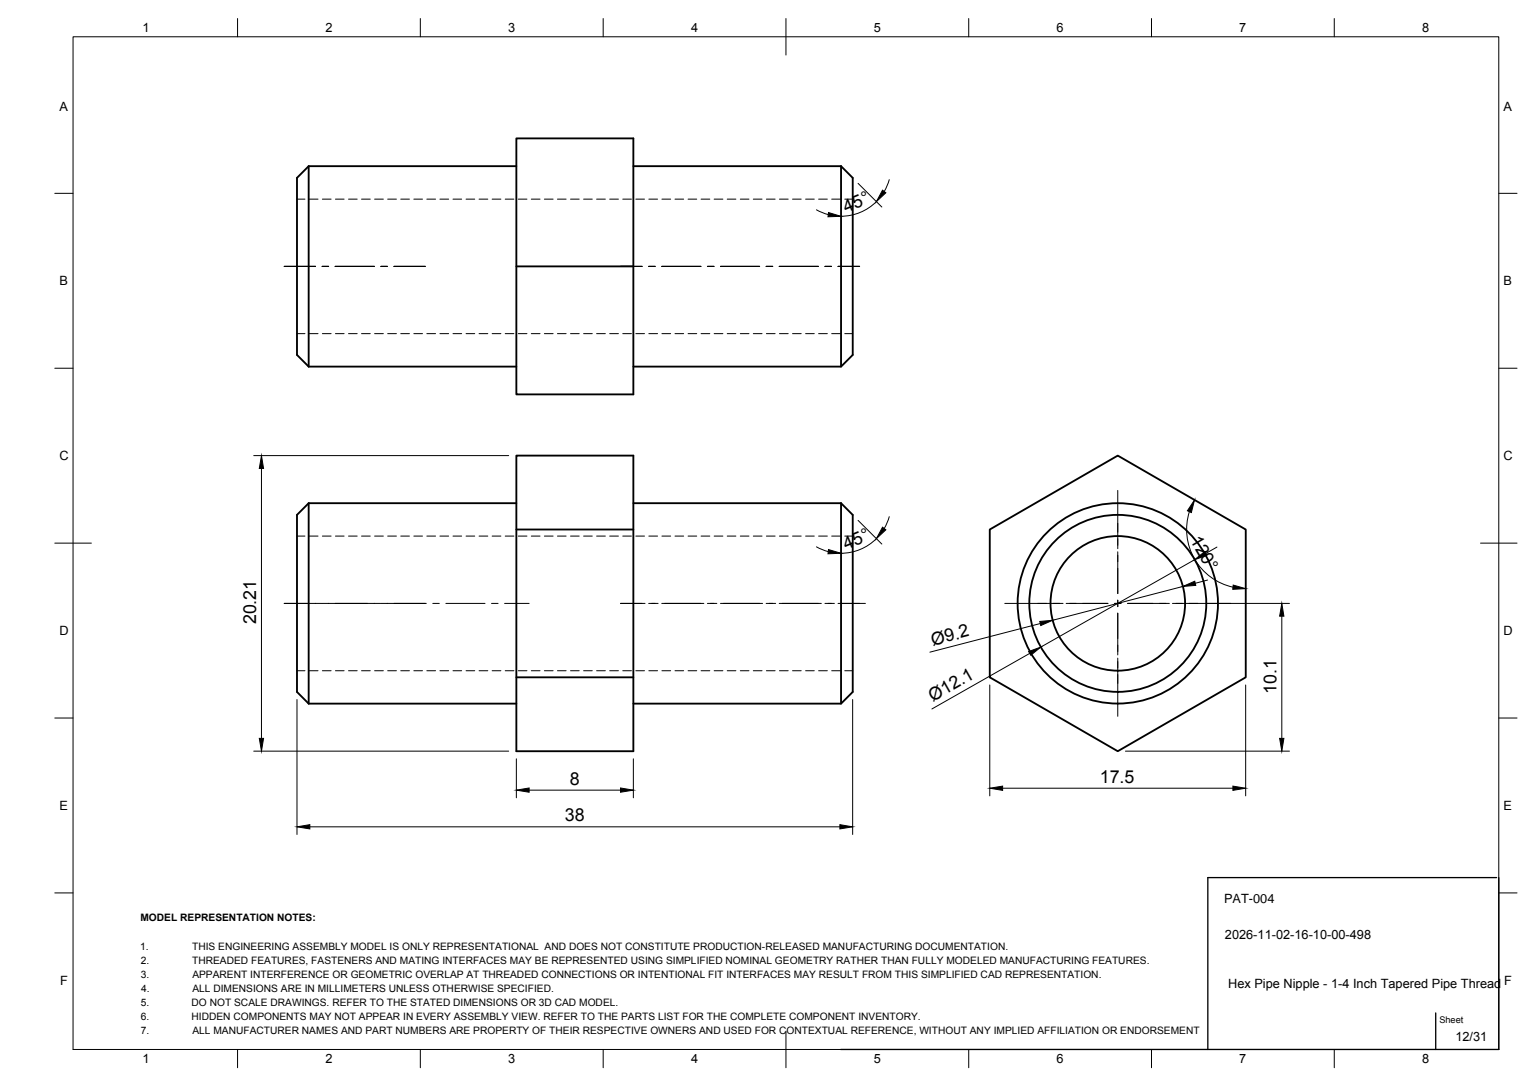
ISO-10303-21;
HEADER;
/* Generated by software containing ST-Developer
 * from STEP Tools, Inc. (www.steptools.com) 
 */

FILE_DESCRIPTION(
/* description */ ('Air blow-off nozzle station'),
/* implementation_level */ '2;1');

FILE_NAME(
/* name */ 'Hex Pipe Nipple - 1-4 Inch Tapered Pipe Thread.step',
/* time_stamp */ '2026-10-27T10:53:54-07:00',
/* author */ (''),
/* organization */ (''),
/* preprocessor_version */ 'ST-DEVELOPER v20.2',
/* originating_system */ 'Autodesk Translation Framework v15.17.0.0',
/* authorisation */ '');

FILE_SCHEMA (('AUTOMOTIVE_DESIGN { 1 0 10303 214 3 1 1 }'));
ENDSEC;

DATA;
#10=MECHANICAL_DESIGN_GEOMETRIC_PRESENTATION_REPRESENTATION('',(#250),#7897);
#163=CONICAL_SURFACE('',#4876,0.645,0.785398163397448);
#164=CONICAL_SURFACE('',#4879,0.645,0.785398163397448);
#200=SHAPE_REPRESENTATION_RELATIONSHIP('SRR','None',#8014,#225);
#225=ADVANCED_BREP_SHAPE_REPRESENTATION('',(#273),#7881);
#250=STYLED_ITEM('',(#8213),#273);
#273=MANIFOLD_SOLID_BREP('Body1',#4301);
#331=FACE_BOUND('',#1013,.T.);
#332=FACE_BOUND('',#1015,.T.);
#333=FACE_BOUND('',#1024,.T.);
#334=FACE_BOUND('',#1029,.T.);
#494=PLANE('',#4861);
#495=PLANE('',#4863);
#496=PLANE('',#4865);
#497=PLANE('',#4866);
#498=PLANE('',#4867);
#499=PLANE('',#4868);
#500=PLANE('',#4869);
#501=PLANE('',#4870);
#502=PLANE('',#4873);
#503=PLANE('',#4881);
#710=FACE_OUTER_BOUND('',#1012,.T.);
#711=FACE_OUTER_BOUND('',#1014,.T.);
#712=FACE_OUTER_BOUND('',#1016,.T.);
#713=FACE_OUTER_BOUND('',#1017,.T.);
#714=FACE_OUTER_BOUND('',#1018,.T.);
#715=FACE_OUTER_BOUND('',#1019,.T.);
#716=FACE_OUTER_BOUND('',#1020,.T.);
#717=FACE_OUTER_BOUND('',#1021,.T.);
#718=FACE_OUTER_BOUND('',#1022,.T.);
#719=FACE_OUTER_BOUND('',#1023,.T.);
#720=FACE_OUTER_BOUND('',#1025,.T.);
#721=FACE_OUTER_BOUND('',#1026,.T.);
#722=FACE_OUTER_BOUND('',#1027,.T.);
#723=FACE_OUTER_BOUND('',#1028,.T.);
#724=FACE_OUTER_BOUND('',#1030,.T.);
#1012=EDGE_LOOP('',(#3663,#3664,#3665,#3666,#3667,#3668));
#1013=EDGE_LOOP('',(#3669));
#1014=EDGE_LOOP('',(#3670,#3671,#3672,#3673,#3674,#3675));
#1015=EDGE_LOOP('',(#3676));
#1016=EDGE_LOOP('',(#3677,#3678,#3679,#3680));
#1017=EDGE_LOOP('',(#3681,#3682,#3683,#3684));
#1018=EDGE_LOOP('',(#3685,#3686,#3687,#3688));
#1019=EDGE_LOOP('',(#3689,#3690,#3691,#3692));
#1020=EDGE_LOOP('',(#3693,#3694,#3695,#3696));
#1021=EDGE_LOOP('',(#3697,#3698,#3699,#3700));
#1022=EDGE_LOOP('',(#3701,#3702,#3703,#3704));
#1023=EDGE_LOOP('',(#3705));
#1024=EDGE_LOOP('',(#3706));
#1025=EDGE_LOOP('',(#3707,#3708,#3709,#3710));
#1026=EDGE_LOOP('',(#3711,#3712,#3713,#3714));
#1027=EDGE_LOOP('',(#3715,#3716,#3717,#3718));
#1028=EDGE_LOOP('',(#3719));
#1029=EDGE_LOOP('',(#3720));
#1030=EDGE_LOOP('',(#3721,#3722,#3723,#3724));
#1419=LINE('',#7451,#1773);
#1420=LINE('',#7453,#1774);
#1421=LINE('',#7455,#1775);
#1422=LINE('',#7457,#1776);
#1423=LINE('',#7459,#1777);
#1424=LINE('',#7460,#1778);
#1425=LINE('',#7466,#1779);
#1426=LINE('',#7468,#1780);
#1427=LINE('',#7470,#1781);
#1428=LINE('',#7472,#1782);
#1429=LINE('',#7474,#1783);
#1430=LINE('',#7475,#1784);
#1431=LINE('',#7479,#1785);
#1432=LINE('',#7480,#1786);
#1433=LINE('',#7482,#1787);
#1434=LINE('',#7484,#1788);
#1435=LINE('',#7486,#1789);
#1436=LINE('',#7488,#1790);
#1437=LINE('',#7492,#1791);
#1438=LINE('',#7500,#1792);
#1439=LINE('',#7504,#1793);
#1440=LINE('',#7508,#1794);
#1441=LINE('',#7513,#1795);
#1773=VECTOR('',#5899,1.);
#1774=VECTOR('',#5900,1.);
#1775=VECTOR('',#5901,1.);
#1776=VECTOR('',#5902,1.);
#1777=VECTOR('',#5903,1.);
#1778=VECTOR('',#5904,1.);
#1779=VECTOR('',#5909,1.);
#1780=VECTOR('',#5910,1.);
#1781=VECTOR('',#5911,1.);
#1782=VECTOR('',#5912,1.);
#1783=VECTOR('',#5913,1.);
#1784=VECTOR('',#5914,1.);
#1785=VECTOR('',#5919,1.);
#1786=VECTOR('',#5920,1.);
#1787=VECTOR('',#5923,1.);
#1788=VECTOR('',#5926,1.);
#1789=VECTOR('',#5929,1.);
#1790=VECTOR('',#5932,1.);
#1791=VECTOR('',#5937,0.685);
#1792=VECTOR('',#5948,0.645);
#1793=VECTOR('',#5953,0.685);
#1794=VECTOR('',#5958,0.645);
#1795=VECTOR('',#5965,0.46);
#1932=CIRCLE('',#4862,0.685);
#1933=CIRCLE('',#4864,0.685);
#1934=CIRCLE('',#4872,0.685);
#1935=CIRCLE('',#4874,0.605);
#1936=CIRCLE('',#4875,0.46);
#1937=CIRCLE('',#4878,0.685);
#1938=CIRCLE('',#4880,0.605);
#1939=CIRCLE('',#4882,0.46);
#2264=VERTEX_POINT('',#7449);
#2265=VERTEX_POINT('',#7450);
#2266=VERTEX_POINT('',#7452);
#2267=VERTEX_POINT('',#7454);
#2268=VERTEX_POINT('',#7456);
#2269=VERTEX_POINT('',#7458);
#2270=VERTEX_POINT('',#7461);
#2271=VERTEX_POINT('',#7464);
#2272=VERTEX_POINT('',#7465);
#2273=VERTEX_POINT('',#7467);
#2274=VERTEX_POINT('',#7469);
#2275=VERTEX_POINT('',#7471);
#2276=VERTEX_POINT('',#7473);
#2277=VERTEX_POINT('',#7476);
#2278=VERTEX_POINT('',#7491);
#2279=VERTEX_POINT('',#7495);
#2280=VERTEX_POINT('',#7497);
#2281=VERTEX_POINT('',#7502);
#2282=VERTEX_POINT('',#7506);
#2283=VERTEX_POINT('',#7510);
#2749=EDGE_CURVE('',#2264,#2265,#1419,.T.);
#2750=EDGE_CURVE('',#2265,#2266,#1420,.T.);
#2751=EDGE_CURVE('',#2266,#2267,#1421,.T.);
#2752=EDGE_CURVE('',#2267,#2268,#1422,.T.);
#2753=EDGE_CURVE('',#2268,#2269,#1423,.T.);
#2754=EDGE_CURVE('',#2269,#2264,#1424,.T.);
#2755=EDGE_CURVE('',#2270,#2270,#1932,.T.);
#2756=EDGE_CURVE('',#2271,#2272,#1425,.T.);
#2757=EDGE_CURVE('',#2272,#2273,#1426,.T.);
#2758=EDGE_CURVE('',#2273,#2274,#1427,.T.);
#2759=EDGE_CURVE('',#2274,#2275,#1428,.T.);
#2760=EDGE_CURVE('',#2275,#2276,#1429,.T.);
#2761=EDGE_CURVE('',#2276,#2271,#1430,.T.);
#2762=EDGE_CURVE('',#2277,#2277,#1933,.T.);
#2763=EDGE_CURVE('',#2271,#2265,#1431,.T.);
#2764=EDGE_CURVE('',#2266,#2276,#1432,.T.);
#2765=EDGE_CURVE('',#2267,#2275,#1433,.T.);
#2766=EDGE_CURVE('',#2268,#2274,#1434,.T.);
#2767=EDGE_CURVE('',#2269,#2273,#1435,.T.);
#2768=EDGE_CURVE('',#2264,#2272,#1436,.T.);
#2769=EDGE_CURVE('',#2277,#2278,#1437,.T.);
#2770=EDGE_CURVE('',#2278,#2278,#1934,.T.);
#2771=EDGE_CURVE('',#2279,#2279,#1935,.T.);
#2772=EDGE_CURVE('',#2280,#2280,#1936,.T.);
#2773=EDGE_CURVE('',#2278,#2279,#1438,.T.);
#2774=EDGE_CURVE('',#2281,#2281,#1937,.T.);
#2775=EDGE_CURVE('',#2281,#2270,#1439,.T.);
#2776=EDGE_CURVE('',#2282,#2282,#1938,.T.);
#2777=EDGE_CURVE('',#2282,#2281,#1440,.T.);
#2778=EDGE_CURVE('',#2283,#2283,#1939,.T.);
#2779=EDGE_CURVE('',#2283,#2280,#1441,.T.);
#3663=ORIENTED_EDGE('',*,*,#2749,.T.);
#3664=ORIENTED_EDGE('',*,*,#2750,.T.);
#3665=ORIENTED_EDGE('',*,*,#2751,.T.);
#3666=ORIENTED_EDGE('',*,*,#2752,.T.);
#3667=ORIENTED_EDGE('',*,*,#2753,.T.);
#3668=ORIENTED_EDGE('',*,*,#2754,.T.);
#3669=ORIENTED_EDGE('',*,*,#2755,.F.);
#3670=ORIENTED_EDGE('',*,*,#2756,.T.);
#3671=ORIENTED_EDGE('',*,*,#2757,.T.);
#3672=ORIENTED_EDGE('',*,*,#2758,.T.);
#3673=ORIENTED_EDGE('',*,*,#2759,.T.);
#3674=ORIENTED_EDGE('',*,*,#2760,.T.);
#3675=ORIENTED_EDGE('',*,*,#2761,.T.);
#3676=ORIENTED_EDGE('',*,*,#2762,.F.);
#3677=ORIENTED_EDGE('',*,*,#2763,.F.);
#3678=ORIENTED_EDGE('',*,*,#2761,.F.);
#3679=ORIENTED_EDGE('',*,*,#2764,.F.);
#3680=ORIENTED_EDGE('',*,*,#2750,.F.);
#3681=ORIENTED_EDGE('',*,*,#2764,.T.);
#3682=ORIENTED_EDGE('',*,*,#2760,.F.);
#3683=ORIENTED_EDGE('',*,*,#2765,.F.);
#3684=ORIENTED_EDGE('',*,*,#2751,.F.);
#3685=ORIENTED_EDGE('',*,*,#2765,.T.);
#3686=ORIENTED_EDGE('',*,*,#2759,.F.);
#3687=ORIENTED_EDGE('',*,*,#2766,.F.);
#3688=ORIENTED_EDGE('',*,*,#2752,.F.);
#3689=ORIENTED_EDGE('',*,*,#2766,.T.);
#3690=ORIENTED_EDGE('',*,*,#2758,.F.);
#3691=ORIENTED_EDGE('',*,*,#2767,.F.);
#3692=ORIENTED_EDGE('',*,*,#2753,.F.);
#3693=ORIENTED_EDGE('',*,*,#2767,.T.);
#3694=ORIENTED_EDGE('',*,*,#2757,.F.);
#3695=ORIENTED_EDGE('',*,*,#2768,.F.);
#3696=ORIENTED_EDGE('',*,*,#2754,.F.);
#3697=ORIENTED_EDGE('',*,*,#2768,.T.);
#3698=ORIENTED_EDGE('',*,*,#2756,.F.);
#3699=ORIENTED_EDGE('',*,*,#2763,.T.);
#3700=ORIENTED_EDGE('',*,*,#2749,.F.);
#3701=ORIENTED_EDGE('',*,*,#2762,.T.);
#3702=ORIENTED_EDGE('',*,*,#2769,.T.);
#3703=ORIENTED_EDGE('',*,*,#2770,.T.);
#3704=ORIENTED_EDGE('',*,*,#2769,.F.);
#3705=ORIENTED_EDGE('',*,*,#2771,.F.);
#3706=ORIENTED_EDGE('',*,*,#2772,.T.);
#3707=ORIENTED_EDGE('',*,*,#2770,.F.);
#3708=ORIENTED_EDGE('',*,*,#2773,.T.);
#3709=ORIENTED_EDGE('',*,*,#2771,.T.);
#3710=ORIENTED_EDGE('',*,*,#2773,.F.);
#3711=ORIENTED_EDGE('',*,*,#2774,.F.);
#3712=ORIENTED_EDGE('',*,*,#2775,.T.);
#3713=ORIENTED_EDGE('',*,*,#2755,.T.);
#3714=ORIENTED_EDGE('',*,*,#2775,.F.);
#3715=ORIENTED_EDGE('',*,*,#2776,.F.);
#3716=ORIENTED_EDGE('',*,*,#2777,.T.);
#3717=ORIENTED_EDGE('',*,*,#2774,.T.);
#3718=ORIENTED_EDGE('',*,*,#2777,.F.);
#3719=ORIENTED_EDGE('',*,*,#2776,.T.);
#3720=ORIENTED_EDGE('',*,*,#2778,.F.);
#3721=ORIENTED_EDGE('',*,*,#2778,.T.);
#3722=ORIENTED_EDGE('',*,*,#2779,.T.);
#3723=ORIENTED_EDGE('',*,*,#2772,.F.);
#3724=ORIENTED_EDGE('',*,*,#2779,.F.);
#3995=CYLINDRICAL_SURFACE('',#4871,0.685);
#3996=CYLINDRICAL_SURFACE('',#4877,0.685);
#3997=CYLINDRICAL_SURFACE('',#4883,0.46);
#4200=ADVANCED_FACE('',(#710,#331),#494,.F.);
#4201=ADVANCED_FACE('',(#711,#332),#495,.T.);
#4202=ADVANCED_FACE('',(#712),#496,.T.);
#4203=ADVANCED_FACE('',(#713),#497,.T.);
#4204=ADVANCED_FACE('',(#714),#498,.T.);
#4205=ADVANCED_FACE('',(#715),#499,.T.);
#4206=ADVANCED_FACE('',(#716),#500,.T.);
#4207=ADVANCED_FACE('',(#717),#501,.T.);
#4208=ADVANCED_FACE('',(#718),#3995,.T.);
#4209=ADVANCED_FACE('',(#719,#333),#502,.T.);
#4210=ADVANCED_FACE('',(#720),#163,.T.);
#4211=ADVANCED_FACE('',(#721),#3996,.T.);
#4212=ADVANCED_FACE('',(#722),#164,.T.);
#4213=ADVANCED_FACE('',(#723,#334),#503,.T.);
#4214=ADVANCED_FACE('',(#724),#3997,.F.);
#4301=CLOSED_SHELL('',(#4200,#4201,#4202,#4203,#4204,#4205,#4206,#4207,
#4208,#4209,#4210,#4211,#4212,#4213,#4214));
#4860=AXIS2_PLACEMENT_3D('',#7447,#5895,#5896);
#4861=AXIS2_PLACEMENT_3D('',#7448,#5897,#5898);
#4862=AXIS2_PLACEMENT_3D('',#7462,#5905,#5906);
#4863=AXIS2_PLACEMENT_3D('',#7463,#5907,#5908);
#4864=AXIS2_PLACEMENT_3D('',#7477,#5915,#5916);
#4865=AXIS2_PLACEMENT_3D('',#7478,#5917,#5918);
#4866=AXIS2_PLACEMENT_3D('',#7481,#5921,#5922);
#4867=AXIS2_PLACEMENT_3D('',#7483,#5924,#5925);
#4868=AXIS2_PLACEMENT_3D('',#7485,#5927,#5928);
#4869=AXIS2_PLACEMENT_3D('',#7487,#5930,#5931);
#4870=AXIS2_PLACEMENT_3D('',#7489,#5933,#5934);
#4871=AXIS2_PLACEMENT_3D('',#7490,#5935,#5936);
#4872=AXIS2_PLACEMENT_3D('',#7493,#5938,#5939);
#4873=AXIS2_PLACEMENT_3D('',#7494,#5940,#5941);
#4874=AXIS2_PLACEMENT_3D('',#7496,#5942,#5943);
#4875=AXIS2_PLACEMENT_3D('',#7498,#5944,#5945);
#4876=AXIS2_PLACEMENT_3D('',#7499,#5946,#5947);
#4877=AXIS2_PLACEMENT_3D('',#7501,#5949,#5950);
#4878=AXIS2_PLACEMENT_3D('',#7503,#5951,#5952);
#4879=AXIS2_PLACEMENT_3D('',#7505,#5954,#5955);
#4880=AXIS2_PLACEMENT_3D('',#7507,#5956,#5957);
#4881=AXIS2_PLACEMENT_3D('',#7509,#5959,#5960);
#4882=AXIS2_PLACEMENT_3D('',#7511,#5961,#5962);
#4883=AXIS2_PLACEMENT_3D('',#7512,#5963,#5964);
#5895=DIRECTION('axis',(0.,0.,1.));
#5896=DIRECTION('refdir',(1.,0.,0.));
#5897=DIRECTION('center_axis',(0.,1.,0.));
#5898=DIRECTION('ref_axis',(1.,0.,0.));
#5899=DIRECTION('',(-0.5,0.,0.866025403784439));
#5900=DIRECTION('',(-1.,0.,-3.29650746237182E-16));
#5901=DIRECTION('',(-0.5,0.,-0.866025403784439));
#5902=DIRECTION('',(0.5,0.,-0.866025403784438));
#5903=DIRECTION('',(1.,0.,0.));
#5904=DIRECTION('',(0.5,0.,0.866025403784439));
#5905=DIRECTION('center_axis',(0.,-1.,0.));
#5906=DIRECTION('ref_axis',(1.,0.,0.));
#5907=DIRECTION('center_axis',(0.,1.,0.));
#5908=DIRECTION('ref_axis',(1.,0.,0.));
#5909=DIRECTION('',(0.5,0.,-0.866025403784439));
#5910=DIRECTION('',(-0.5,0.,-0.866025403784439));
#5911=DIRECTION('',(-1.,0.,0.));
#5912=DIRECTION('',(-0.5,0.,0.866025403784438));
#5913=DIRECTION('',(0.5,0.,0.866025403784439));
#5914=DIRECTION('',(1.,0.,3.29650746237182E-16));
#5915=DIRECTION('center_axis',(0.,1.,0.));
#5916=DIRECTION('ref_axis',(1.,0.,0.));
#5917=DIRECTION('center_axis',(-3.29650746237182E-16,0.,1.));
#5918=DIRECTION('ref_axis',(1.,0.,3.29650746237182E-16));
#5919=DIRECTION('',(0.,-1.,0.));
#5920=DIRECTION('',(0.,1.,0.));
#5921=DIRECTION('center_axis',(-0.866025403784439,0.,0.5));
#5922=DIRECTION('ref_axis',(0.5,0.,0.866025403784439));
#5923=DIRECTION('',(0.,1.,0.));
#5924=DIRECTION('center_axis',(-0.866025403784439,0.,-0.5));
#5925=DIRECTION('ref_axis',(-0.5,0.,0.866025403784439));
#5926=DIRECTION('',(0.,1.,0.));
#5927=DIRECTION('center_axis',(0.,0.,-1.));
#5928=DIRECTION('ref_axis',(-1.,0.,0.));
#5929=DIRECTION('',(0.,1.,0.));
#5930=DIRECTION('center_axis',(0.866025403784439,0.,-0.5));
#5931=DIRECTION('ref_axis',(-0.5,0.,-0.866025403784439));
#5932=DIRECTION('',(0.,1.,0.));
#5933=DIRECTION('center_axis',(0.866025403784439,0.,0.5));
#5934=DIRECTION('ref_axis',(0.5,0.,-0.866025403784439));
#5935=DIRECTION('center_axis',(0.,-1.,0.));
#5936=DIRECTION('ref_axis',(1.,0.,0.));
#5937=DIRECTION('',(0.,1.,0.));
#5938=DIRECTION('center_axis',(0.,-1.,0.));
#5939=DIRECTION('ref_axis',(1.,0.,0.));
#5940=DIRECTION('center_axis',(0.,1.,0.));
#5941=DIRECTION('ref_axis',(0.,0.,1.));
#5942=DIRECTION('center_axis',(0.,-1.,0.));
#5943=DIRECTION('ref_axis',(1.,0.,0.));
#5944=DIRECTION('center_axis',(0.,-1.,0.));
#5945=DIRECTION('ref_axis',(1.,0.,0.));
#5946=DIRECTION('center_axis',(0.,-1.,0.));
#5947=DIRECTION('ref_axis',(1.,0.,0.));
#5948=DIRECTION('',(0.707106781186547,0.707106781186548,8.65956056235493E-17));
#5949=DIRECTION('center_axis',(0.,-1.,0.));
#5950=DIRECTION('ref_axis',(1.,0.,0.));
#5951=DIRECTION('center_axis',(0.,-1.,0.));
#5952=DIRECTION('ref_axis',(1.,0.,0.));
#5953=DIRECTION('',(0.,1.,0.));
#5954=DIRECTION('center_axis',(0.,1.,0.));
#5955=DIRECTION('ref_axis',(1.,0.,0.));
#5956=DIRECTION('center_axis',(0.,-1.,0.));
#5957=DIRECTION('ref_axis',(1.,0.,0.));
#5958=DIRECTION('',(-0.707106781186547,0.707106781186548,-8.65956056235493E-17));
#5959=DIRECTION('center_axis',(0.,-1.,0.));
#5960=DIRECTION('ref_axis',(0.,0.,-1.));
#5961=DIRECTION('center_axis',(0.,-1.,0.));
#5962=DIRECTION('ref_axis',(1.,0.,0.));
#5963=DIRECTION('center_axis',(0.,-1.,0.));
#5964=DIRECTION('ref_axis',(1.,0.,0.));
#5965=DIRECTION('',(0.,1.,0.));
#7447=CARTESIAN_POINT('',(0.,0.,0.));
#7448=CARTESIAN_POINT('Origin',(0.,-0.4,0.));
#7449=CARTESIAN_POINT('',(1.01036297108185,-0.4,0.));
#7450=CARTESIAN_POINT('',(0.505181485540923,-0.4,0.875));
#7451=CARTESIAN_POINT('',(0.505181485540923,-0.4,0.875));
#7452=CARTESIAN_POINT('',(-0.505181485540923,-0.4,0.875));
#7453=CARTESIAN_POINT('',(-0.505181485540923,-0.4,0.875));
#7454=CARTESIAN_POINT('',(-1.01036297108185,-0.4,-1.23733777851239E-16));
#7455=CARTESIAN_POINT('',(-1.01036297108185,-0.4,-1.23733777851239E-16));
#7456=CARTESIAN_POINT('',(-0.505181485540922,-0.4,-0.875));
#7457=CARTESIAN_POINT('',(-0.505181485540922,-0.4,-0.875));
#7458=CARTESIAN_POINT('',(0.505181485540923,-0.4,-0.875));
#7459=CARTESIAN_POINT('',(0.505181485540923,-0.4,-0.875));
#7460=CARTESIAN_POINT('',(1.01036297108185,-0.4,0.));
#7461=CARTESIAN_POINT('',(-0.685,-0.4,-8.38883057415937E-17));
#7462=CARTESIAN_POINT('Origin',(0.,-0.4,0.));
#7463=CARTESIAN_POINT('Origin',(0.,0.4,0.));
#7464=CARTESIAN_POINT('',(0.505181485540923,0.4,0.875));
#7465=CARTESIAN_POINT('',(1.01036297108185,0.4,0.));
#7466=CARTESIAN_POINT('',(0.505181485540923,0.4,0.875));
#7467=CARTESIAN_POINT('',(0.505181485540923,0.4,-0.875));
#7468=CARTESIAN_POINT('',(1.01036297108185,0.4,0.));
#7469=CARTESIAN_POINT('',(-0.505181485540922,0.4,-0.875));
#7470=CARTESIAN_POINT('',(0.505181485540923,0.4,-0.875));
#7471=CARTESIAN_POINT('',(-1.01036297108185,0.4,-1.23733777851239E-16));
#7472=CARTESIAN_POINT('',(-0.505181485540922,0.4,-0.875));
#7473=CARTESIAN_POINT('',(-0.505181485540923,0.4,0.875));
#7474=CARTESIAN_POINT('',(-1.01036297108185,0.4,-1.23733777851239E-16));
#7475=CARTESIAN_POINT('',(-0.505181485540923,0.4,0.875));
#7476=CARTESIAN_POINT('',(-0.685,0.4,8.38883057415937E-17));
#7477=CARTESIAN_POINT('Origin',(0.,0.4,0.));
#7478=CARTESIAN_POINT('Origin',(-0.505181485540923,0.,0.875));
#7479=CARTESIAN_POINT('',(0.505181485540923,0.,0.875));
#7480=CARTESIAN_POINT('',(-0.505181485540923,0.,0.875));
#7481=CARTESIAN_POINT('Origin',(-1.01036297108185,0.,-1.23733777851239E-16));
#7482=CARTESIAN_POINT('',(-1.01036297108185,0.,-1.23733777851239E-16));
#7483=CARTESIAN_POINT('Origin',(-0.505181485540922,0.,-0.875));
#7484=CARTESIAN_POINT('',(-0.505181485540922,0.,-0.875));
#7485=CARTESIAN_POINT('Origin',(0.505181485540923,0.,-0.875));
#7486=CARTESIAN_POINT('',(0.505181485540923,0.,-0.875));
#7487=CARTESIAN_POINT('Origin',(1.01036297108185,0.,0.));
#7488=CARTESIAN_POINT('',(1.01036297108185,0.,0.));
#7489=CARTESIAN_POINT('Origin',(0.505181485540923,0.,0.875));
#7490=CARTESIAN_POINT('Origin',(0.,0.,0.));
#7491=CARTESIAN_POINT('',(-0.685,1.82,-8.38883057415937E-17));
#7492=CARTESIAN_POINT('',(-0.685,0.,-8.38883057415937E-17));
#7493=CARTESIAN_POINT('Origin',(0.,1.82,0.));
#7494=CARTESIAN_POINT('Origin',(0.605,1.9,0.));
#7495=CARTESIAN_POINT('',(-0.605,1.9,-7.40911313484149E-17));
#7496=CARTESIAN_POINT('Origin',(0.,1.9,0.));
#7497=CARTESIAN_POINT('',(-0.46,1.9,-5.63337527607782E-17));
#7498=CARTESIAN_POINT('Origin',(0.,1.9,0.));
#7499=CARTESIAN_POINT('Origin',(0.,1.86,0.));
#7500=CARTESIAN_POINT('',(-0.645,1.86,-7.89897185450043E-17));
#7501=CARTESIAN_POINT('Origin',(0.,0.,0.));
#7502=CARTESIAN_POINT('',(-0.685,-1.82,-8.38883057415937E-17));
#7503=CARTESIAN_POINT('Origin',(0.,-1.82,0.));
#7504=CARTESIAN_POINT('',(-0.685,0.,-8.38883057415937E-17));
#7505=CARTESIAN_POINT('Origin',(0.,-1.86,0.));
#7506=CARTESIAN_POINT('',(-0.605,-1.9,-7.40911313484149E-17));
#7507=CARTESIAN_POINT('Origin',(0.,-1.9,0.));
#7508=CARTESIAN_POINT('',(-0.645,-1.86,-7.89897185450043E-17));
#7509=CARTESIAN_POINT('Origin',(0.46,-1.9,0.));
#7510=CARTESIAN_POINT('',(-0.46,-1.9,-5.63337527607782E-17));
#7511=CARTESIAN_POINT('Origin',(0.,-1.9,0.));
#7512=CARTESIAN_POINT('Origin',(0.,0.,0.));
#7513=CARTESIAN_POINT('',(-0.46,0.,-5.63337527607782E-17));
#7849=UNCERTAINTY_MEASURE_WITH_UNIT(LENGTH_MEASURE(0.001),#7898,
'DISTANCE_ACCURACY_VALUE',
'Maximum model space distance between geometric entities at asserted c
onnectivities');
#7865=UNCERTAINTY_MEASURE_WITH_UNIT(LENGTH_MEASURE(0.001),#7898,
'DISTANCE_ACCURACY_VALUE',
'Maximum model space distance between geometric entities at asserted c
onnectivities');
#7881=(
GEOMETRIC_REPRESENTATION_CONTEXT(3)
GLOBAL_UNCERTAINTY_ASSIGNED_CONTEXT((#7849))
GLOBAL_UNIT_ASSIGNED_CONTEXT((#7898,#7900,#7901))
REPRESENTATION_CONTEXT('','3D')
);
#7897=(
GEOMETRIC_REPRESENTATION_CONTEXT(3)
GLOBAL_UNCERTAINTY_ASSIGNED_CONTEXT((#7865))
GLOBAL_UNIT_ASSIGNED_CONTEXT((#7898,#7900,#7901))
REPRESENTATION_CONTEXT('','3D')
);
#7898=(
LENGTH_UNIT()
NAMED_UNIT(*)
SI_UNIT(.CENTI.,.METRE.)
);
#7900=(
NAMED_UNIT(*)
PLANE_ANGLE_UNIT()
SI_UNIT($,.RADIAN.)
);
#7901=(
NAMED_UNIT(*)
SI_UNIT($,.STERADIAN.)
SOLID_ANGLE_UNIT()
);
#7917=SHAPE_DEFINITION_REPRESENTATION(#7948,#8014);
#7948=PRODUCT_DEFINITION_SHAPE('',$,#8046);
#8014=SHAPE_REPRESENTATION('',(#4860),#7881);
#8030=PRODUCT_DEFINITION_CONTEXT('part definition',#8125,'design');
#8046=PRODUCT_DEFINITION(
'Hex Pipe Nipple - 1-4 Inch Tapered Pipe Thread',
'Hex Pipe Nipple - 1-4 Inch Tapered Pipe Thread',#8077,#8030);
#8077=PRODUCT_DEFINITION_FORMATION('',$,#8142);
#8125=APPLICATION_CONTEXT(
'Core Data for Automotive Mechanical Design Process');
#8126=PRODUCT_CONTEXT('part definition',#8125,'mechanical');
#8142=PRODUCT('Hex Pipe Nipple - 1-4 Inch Tapered Pipe Thread',
'Hex Pipe Nipple - 1-4 Inch Tapered Pipe Thread',
'Hex Pipe Nipple - 1-4 Inch Tapered Pipe Thread',(#8126));
#8207=COLOUR_RGB('Sky Blue',0.24,0.69,0.87);
#8208=FILL_AREA_STYLE_COLOUR('',#8207);
#8209=FILL_AREA_STYLE('',(#8208));
#8210=SURFACE_STYLE_FILL_AREA(#8209);
#8211=SURFACE_SIDE_STYLE('',(#8210));
#8212=SURFACE_STYLE_USAGE(.BOTH.,#8211);
#8213=PRESENTATION_STYLE_ASSIGNMENT((#8212));
ENDSEC;
END-ISO-10303-21;
